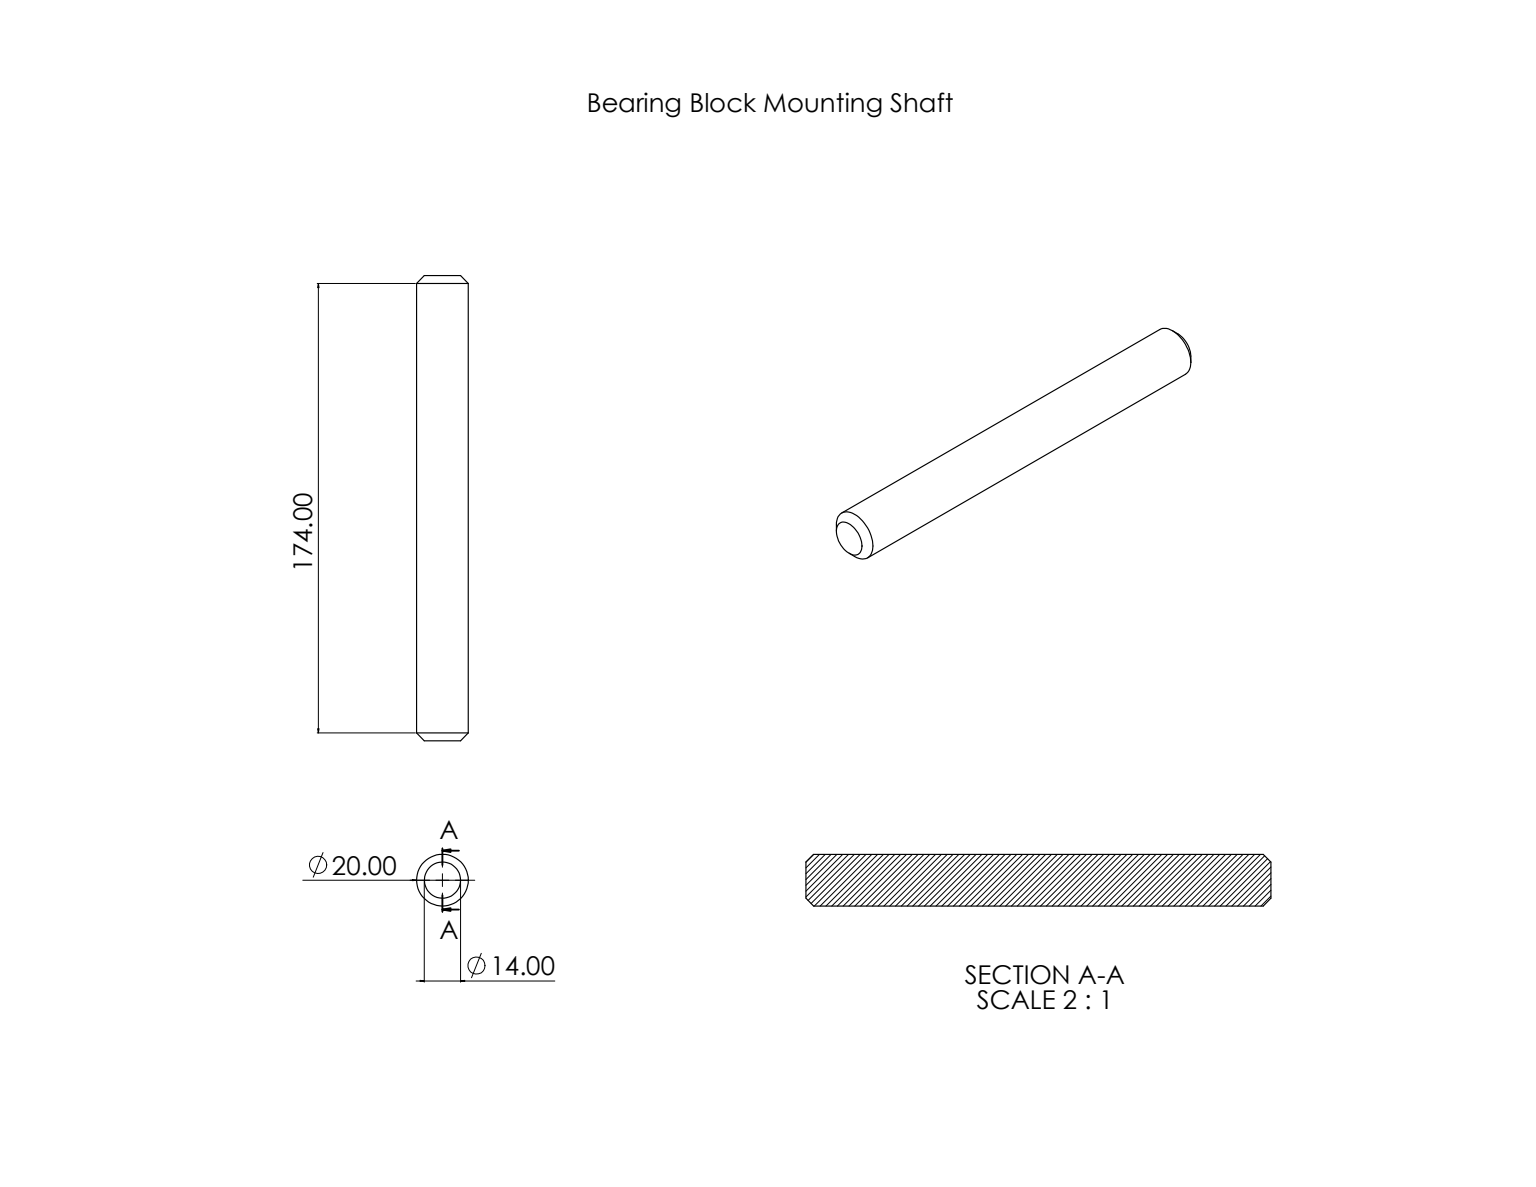
ISO-10303-21;
HEADER;
FILE_DESCRIPTION (('STEP AP214'),
    '1' );
FILE_NAME ('Bearing Block Mounting Shaft.step',
    '2026-10-19T17:36:30',
    ( '' ),
    ( '' ),
    'SwSTEP 2.0',
    'SolidWorks 2025',
    '' );
FILE_SCHEMA (( 'AUTOMOTIVE_DESIGN' ));
ENDSEC;

DATA;
#28=EDGE_CURVE ( 'NONE', #7100, #9959, #2772, .T. ) ;
#57=FACE_OUTER_BOUND ( 'NONE', #633, .T. ) ;
#142=AXIS2_PLACEMENT_3D ( 'NONE', #1198, #5064, #7978 ) ;
#156=DIRECTION ( 'NONE',  ( 1.000000000000000000, 0.000000000000000000, 0.000000000000000000 ) ) ;
#168=DIRECTION ( 'NONE',  ( 0.000000000000000000, -0.000000000000000000, -1.000000000000000000 ) ) ;
#207=DIRECTION ( 'NONE',  ( 1.000000000000000000, 0.000000000000000000, 0.000000000000000000 ) ) ;
#243=EDGE_CURVE ( 'NONE', #9959, #918, #9739, .T. ) ;
#295=DIRECTION ( 'NONE',  ( 1.000000000000000000, 0.000000000000000000, 0.000000000000000000 ) ) ;
#366=ORIENTED_EDGE ( 'NONE', *, *, #12537, .F. ) ;
#595=CIRCLE ( 'NONE', #1008, 10.00000000000000355 ) ;
#633=EDGE_LOOP ( 'NONE', ( #366, #4722, #9019, #2561 ) ) ;
#785=AXIS2_PLACEMENT_3D ( 'NONE', #3854, #7731, #7665 ) ;
#812=PLANE ( 'NONE',  #785 ) ;
#909=( LENGTH_UNIT ( ) NAMED_UNIT ( * ) SI_UNIT ( .MILLI., .METRE. ) );
#918=VERTEX_POINT ( 'NONE', #1888 ) ;
#923=STYLED_ITEM('',(#12584),#10571);
#1001=UNCERTAINTY_MEASURE_WITH_UNIT (LENGTH_MEASURE( 1.000000000000000082E-05 ), #909, 'distance_accuracy_value', 'NONE');
#1008=AXIS2_PLACEMENT_3D ( 'NONE', #4470, #7262, #4286 ) ;
#1021=SHAPE_DEFINITION_REPRESENTATION ( #9949, #1739 ) ;
#1198=CARTESIAN_POINT ( 'NONE',  ( 0.000000000000000000, 20.00000000000000355, 109.9999999999999858 ) ) ;
#1226=DIRECTION ( 'NONE',  ( -0.7071067811865469066, 0.000000000000000000, -0.7071067811865482389 ) ) ;
#1295=DIRECTION ( 'NONE',  ( -0.7071067811865502373, 8.659560562354966138E-17, 0.7071067811865449082 ) ) ;
#1363=ORIENTED_EDGE ( 'NONE', *, *, #3044, .T. ) ;
#1376=ORIENTED_EDGE ( 'NONE', *, *, #2334, .F. ) ;
#1391=ORIENTED_EDGE ( 'NONE', *, *, #2650, .F. ) ;
#1488=AXIS2_PLACEMENT_3D ( 'NONE', #10254, #5256, #5445 ) ;
#1523=EDGE_LOOP ( 'NONE', ( #7715, #1363 ) ) ;
#1633=EDGE_LOOP ( 'NONE', ( #1376, #9658, #7352, #7644 ) ) ;
#1682=DIRECTION ( 'NONE',  ( 1.000000000000000000, 0.000000000000000000, 0.000000000000000000 ) ) ;
#1688=CIRCLE ( 'NONE', #1488, 10.00000000000000355 ) ;
#1693=EDGE_CURVE ( 'NONE', #9959, #2943, #595, .T. ) ;
#1721=APPLICATION_CONTEXT ( 'automotive_design' ) ;
#1739=SHAPE_REPRESENTATION ( 'Bearing Block Mounting Shaft', ( #9021 ), #11237 ) ;
#1777=ORIENTED_EDGE ( 'NONE', *, *, #28, .F. ) ;
#1780=ORIENTED_EDGE ( 'NONE', *, *, #11066, .F. ) ;
#1782=AXIS2_PLACEMENT_3D ( 'NONE', #11582, #168, #295 ) ;
#1878=VERTEX_POINT ( 'NONE', #7643 ) ;
#1888=CARTESIAN_POINT ( 'NONE',  ( 10.00000000000000355, 20.00000000000000355, 106.9999999999999574 ) ) ;
#1955=DIRECTION ( 'NONE',  ( 1.000000000000000000, 0.000000000000000000, 0.000000000000000000 ) ) ;
#2154=CONICAL_SURFACE ( 'NONE', #142, 6.999999999999978684, 0.7853981633974473908 ) ;
#2218=ORIENTED_EDGE ( 'NONE', *, *, #4435, .F. ) ;
#2219=DIRECTION ( 'NONE',  ( 0.7071067811865469066, 8.659560562354926695E-17, -0.7071067811865482389 ) ) ;
#2235=EDGE_CURVE ( 'NONE', #7100, #3380, #7707, .T. ) ;
#2328=CARTESIAN_POINT ( 'NONE',  ( 10.00000000000000355, 20.00000000000000355, -66.99999999999998579 ) ) ;
#2334=EDGE_CURVE ( 'NONE', #3380, #2943, #7056, .T. ) ;
#2472=EDGE_LOOP ( 'NONE', ( #3080, #8282, #4849, #12524 ) ) ;
#2561=ORIENTED_EDGE ( 'NONE', *, *, #2650, .T. ) ;
#2616=VECTOR ( 'NONE', #8531, 1000.000000000000000 ) ;
#2650=EDGE_CURVE ( 'NONE', #918, #9719, #3640, .T. ) ;
#2700=FACE_OUTER_BOUND ( 'NONE', #8576, .T. ) ;
#2727=VECTOR ( 'NONE', #6543, 1000.000000000000000 ) ;
#2744=DIRECTION ( 'NONE',  ( 0.000000000000000000, 0.000000000000000000, 1.000000000000000000 ) ) ;
#2772=LINE ( 'NONE', #2328, #9517 ) ;
#2910=CARTESIAN_POINT ( 'NONE',  ( 0.000000000000000000, 20.00000000000000355, -70.00000000000000000 ) ) ;
#2943=VERTEX_POINT ( 'NONE', #4688 ) ;
#3044=EDGE_CURVE ( 'NONE', #8530, #1878, #4880, .T. ) ;
#3080=ORIENTED_EDGE ( 'NONE', *, *, #1693, .T. ) ;
#3085=DIRECTION ( 'NONE',  ( 0.7071067811865502373, 0.000000000000000000, 0.7071067811865449082 ) ) ;
#3105=ADVANCED_FACE ( 'NONE', ( #57 ), #4878, .T. ) ;
#3203=PRODUCT_DEFINITION_CONTEXT ( 'detailed design', #9995, 'design' ) ;
#3380=VERTEX_POINT ( 'NONE', #8422 ) ;
#3429=ORIENTED_EDGE ( 'NONE', *, *, #2334, .T. ) ;
#3453=FACE_OUTER_BOUND ( 'NONE', #2472, .T. ) ;
#3481=CARTESIAN_POINT ( 'NONE',  ( 6.999999999999978684, 20.00000000000000355, 109.9999999999999858 ) ) ;
#3486=CARTESIAN_POINT ( 'NONE',  ( 0.000000000000000000, 20.00000000000000355, 109.9999999999999858 ) ) ;
#3549=AXIS2_PLACEMENT_3D ( 'NONE', #6623, #4604, #1682 ) ;
#3564=ORIENTED_EDGE ( 'NONE', *, *, #10628, .F. ) ;
#3565=LINE ( 'NONE', #6666, #2727 ) ;
#3640=CIRCLE ( 'NONE', #10729, 10.00000000000000355 ) ;
#3657=ORIENTED_EDGE ( 'NONE', *, *, #4358, .T. ) ;
#3680=EDGE_LOOP ( 'NONE', ( #12031, #12477 ) ) ;
#3741=( GEOMETRIC_REPRESENTATION_CONTEXT ( 3 ) GLOBAL_UNCERTAINTY_ASSIGNED_CONTEXT ( ( #1001 ) ) GLOBAL_UNIT_ASSIGNED_CONTEXT ( ( #909, #4778, #8708 ) ) REPRESENTATION_CONTEXT ( 'NONE', 'WORKASPACE' ) );
#3783=ADVANCED_FACE ( 'NONE', ( #10854 ), #4479, .T. ) ;
#3801=AXIS2_PLACEMENT_3D ( 'NONE', #3486, #12431, #11475 ) ;
#3854=CARTESIAN_POINT ( 'NONE',  ( 0.000000000000000000, 0.000000000000000000, -70.00000000000000000 ) ) ;
#3872=DIRECTION ( 'NONE',  ( 0.000000000000000000, 0.000000000000000000, -1.000000000000000000 ) ) ;
#3876=SHAPE_REPRESENTATION_RELATIONSHIP ( 'NONE' , 'NONE' ,  #1739, #11260 ) ;
#4060=CARTESIAN_POINT ( 'NONE',  ( 0.000000000000000000, 20.00000000000000355, 106.9999999999999574 ) ) ;
#4063=CARTESIAN_POINT ( 'NONE',  ( 0.000000000000000000, 20.00000000000000355, -66.99999999999998579 ) ) ;
#4130=( LENGTH_UNIT ( ) NAMED_UNIT ( * ) SI_UNIT ( .MILLI., .METRE. ) );
#4202=ADVANCED_FACE ( 'NONE', ( #5586 ), #10493, .T. ) ;
#4286=DIRECTION ( 'NONE',  ( 1.000000000000000000, 0.000000000000000000, 0.000000000000000000 ) ) ;
#4357=CARTESIAN_POINT ( 'NONE',  ( 6.999999999999964473, 20.00000000000000355, -70.00000000000000000 ) ) ;
#4358=EDGE_CURVE ( 'NONE', #8530, #918, #11030, .T. ) ;
#4361=CONICAL_SURFACE ( 'NONE', #8417, 10.00000000000000355, 0.7853981633974520538 ) ;
#4397=DIRECTION ( 'NONE',  ( 0.000000000000000000, 0.000000000000000000, 1.000000000000000000 ) ) ;
#4415=FACE_OUTER_BOUND ( 'NONE', #1523, .T. ) ;
#4435=EDGE_CURVE ( 'NONE', #3380, #7100, #5240, .T. ) ;
#4470=CARTESIAN_POINT ( 'NONE',  ( 0.000000000000000000, 20.00000000000000355, -66.99999999999998579 ) ) ;
#4479=CONICAL_SURFACE ( 'NONE', #6106, 10.00000000000000355, 0.7853981633974520538 ) ;
#4601=CIRCLE ( 'NONE', #12299, 6.999999999999978684 ) ;
#4604=DIRECTION ( 'NONE',  ( 0.000000000000000000, 0.000000000000000000, -1.000000000000000000 ) ) ;
#4662=CARTESIAN_POINT ( 'NONE',  ( 10.00000000000000355, 20.00000000000000355, -70.00000000000000000 ) ) ;
#4688=CARTESIAN_POINT ( 'NONE',  ( -10.00000000000000355, 20.00000000000000355, -66.99999999999998579 ) ) ;
#4722=ORIENTED_EDGE ( 'NONE', *, *, #6731, .T. ) ;
#4740=PRODUCT_DEFINITION_FORMATION_WITH_SPECIFIED_SOURCE ( 'ANY', '', #5086, .NOT_KNOWN. ) ;
#4778=( NAMED_UNIT ( * ) PLANE_ANGLE_UNIT ( ) SI_UNIT ( $, .RADIAN. ) );
#4849=ORIENTED_EDGE ( 'NONE', *, *, #11066, .T. ) ;
#4878=CYLINDRICAL_SURFACE ( 'NONE', #5286, 10.00000000000000355 ) ;
#4880=CIRCLE ( 'NONE', #10737, 6.999999999999978684 ) ;
#5026=( NAMED_UNIT ( * ) SI_UNIT ( $, .STERADIAN. ) SOLID_ANGLE_UNIT ( ) );
#5064=DIRECTION ( 'NONE',  ( 0.000000000000000000, 0.000000000000000000, -1.000000000000000000 ) ) ;
#5086=PRODUCT ( 'Bearing Block Mounting Shaft', 'Bearing Block Mounting Shaft', '', ( #9769 ) ) ;
#5216=AXIS2_PLACEMENT_3D ( 'NONE', #8293, #7331, #8044 ) ;
#5240=CIRCLE ( 'NONE', #1782, 6.999999999999964473 ) ;
#5256=DIRECTION ( 'NONE',  ( -0.000000000000000000, -0.000000000000000000, 1.000000000000000000 ) ) ;
#5286=AXIS2_PLACEMENT_3D ( 'NONE', #2910, #8871, #1955 ) ;
#5361=ADVANCED_FACE ( 'NONE', ( #8614 ), #812, .F. ) ;
#5438=PRODUCT_DEFINITION ( 'UNKNOWN', '', #4740, #3203 ) ;
#5445=DIRECTION ( 'NONE',  ( 1.000000000000000000, 0.000000000000000000, 0.000000000000000000 ) ) ;
#5488=VECTOR ( 'NONE', #1295, 1000.000000000000114 ) ;
#5515=CARTESIAN_POINT ( 'NONE',  ( 0.000000000000000000, 20.00000000000000355, 109.9999999999999858 ) ) ;
#5586=FACE_OUTER_BOUND ( 'NONE', #8684, .T. ) ;
#5661=ORIENTED_EDGE ( 'NONE', *, *, #3044, .F. ) ;
#6036=DIRECTION ( 'NONE',  ( -0.000000000000000000, -0.000000000000000000, 1.000000000000000000 ) ) ;
#6063=CLOSED_SHELL ( 'NONE', ( #11041, #9772, #7585, #3105, #5361, #10436, #4202, #3783 ) ) ;
#6106=AXIS2_PLACEMENT_3D ( 'NONE', #4063, #6036, #9910 ) ;
#6169=CARTESIAN_POINT ( 'NONE',  ( -6.999999999999978684, 20.00000000000000355, 109.9999999999999858 ) ) ;
#6543=DIRECTION ( 'NONE',  ( 0.000000000000000000, 0.000000000000000000, 1.000000000000000000 ) ) ;
#6578=DIRECTION ( 'NONE',  ( -0.000000000000000000, 0.000000000000000000, 1.000000000000000000 ) ) ;
#6623=CARTESIAN_POINT ( 'NONE',  ( 0.000000000000000000, 20.00000000000000355, 106.9999999999999574 ) ) ;
#6666=CARTESIAN_POINT ( 'NONE',  ( -10.00000000000000355, 20.00000000000000355, -70.00000000000000000 ) ) ;
#6689=DIRECTION ( 'NONE',  ( 1.000000000000000000, 0.000000000000000000, 0.000000000000000000 ) ) ;
#6731=EDGE_CURVE ( 'NONE', #2943, #9959, #1688, .T. ) ;
#6742=DIRECTION ( 'NONE',  ( 0.000000000000000000, -0.000000000000000000, -1.000000000000000000 ) ) ;
#6922=LINE ( 'NONE', #6169, #10632 ) ;
#7056=LINE ( 'NONE', #9985, #5488 ) ;
#7100=VERTEX_POINT ( 'NONE', #4357 ) ;
#7169=ORIENTED_EDGE ( 'NONE', *, *, #10215, .F. ) ;
#7262=DIRECTION ( 'NONE',  ( -0.000000000000000000, -0.000000000000000000, 1.000000000000000000 ) ) ;
#7331=DIRECTION ( 'NONE',  ( -0.000000000000000000, 0.000000000000000000, 1.000000000000000000 ) ) ;
#7352=ORIENTED_EDGE ( 'NONE', *, *, #28, .T. ) ;
#7482=ORIENTED_EDGE ( 'NONE', *, *, #4358, .F. ) ;
#7585=ADVANCED_FACE ( 'NONE', ( #3453 ), #10120, .T. ) ;
#7643=CARTESIAN_POINT ( 'NONE',  ( -6.999999999999978684, 20.00000000000000355, 109.9999999999999858 ) ) ;
#7644=ORIENTED_EDGE ( 'NONE', *, *, #6731, .F. ) ;
#7665=DIRECTION ( 'NONE',  ( 1.000000000000000000, 0.000000000000000000, 0.000000000000000000 ) ) ;
#7707=CIRCLE ( 'NONE', #8317, 6.999999999999964473 ) ;
#7715=ORIENTED_EDGE ( 'NONE', *, *, #10215, .T. ) ;
#7731=DIRECTION ( 'NONE',  ( -0.000000000000000000, 0.000000000000000000, 1.000000000000000000 ) ) ;
#7800=MECHANICAL_DESIGN_GEOMETRIC_PRESENTATION_REPRESENTATION('',(#923),#3741);
#7938=DIRECTION ( 'NONE',  ( 1.000000000000000000, 0.000000000000000000, 0.000000000000000000 ) ) ;
#7978=DIRECTION ( 'NONE',  ( -1.000000000000000000, 0.000000000000000000, 0.000000000000000000 ) ) ;
#8036=ORIENTED_EDGE ( 'NONE', *, *, #10628, .T. ) ;
#8042=CARTESIAN_POINT ( 'NONE',  ( -10.00000000000000355, 20.00000000000000355, 106.9999999999999574 ) ) ;
#8044=DIRECTION ( 'NONE',  ( 1.000000000000000000, 0.000000000000000000, 0.000000000000000000 ) ) ;
#8116=CARTESIAN_POINT ( 'NONE',  ( 6.999999999999978684, 20.00000000000000355, 109.9999999999999858 ) ) ;
#8195=AXIS2_PLACEMENT_3D ( 'NONE', #12083, #4397, #12144 ) ;
#8282=ORIENTED_EDGE ( 'NONE', *, *, #12537, .T. ) ;
#8293=CARTESIAN_POINT ( 'NONE',  ( 0.000000000000000000, 0.000000000000000000, 109.9999999999999858 ) ) ;
#8317=AXIS2_PLACEMENT_3D ( 'NONE', #9862, #6742, #156 ) ;
#8374=DIRECTION ( 'NONE',  ( 1.000000000000000000, 0.000000000000000000, 0.000000000000000000 ) ) ;
#8417=AXIS2_PLACEMENT_3D ( 'NONE', #9434, #10494, #6689 ) ;
#8422=CARTESIAN_POINT ( 'NONE',  ( -6.999999999999964473, 20.00000000000000355, -70.00000000000000000 ) ) ;
#8497=DIRECTION ( 'NONE',  ( -0.000000000000000000, 0.000000000000000000, 1.000000000000000000 ) ) ;
#8530=VERTEX_POINT ( 'NONE', #3481 ) ;
#8531=DIRECTION ( 'NONE',  ( 0.000000000000000000, 0.000000000000000000, 1.000000000000000000 ) ) ;
#8576=EDGE_LOOP ( 'NONE', ( #2218, #3429, #10393, #1777 ) ) ;
#8614=FACE_OUTER_BOUND ( 'NONE', #3680, .T. ) ;
#8684=EDGE_LOOP ( 'NONE', ( #7482, #7169, #8036, #1391 ) ) ;
#8686=UNCERTAINTY_MEASURE_WITH_UNIT (LENGTH_MEASURE( 1.000000000000000082E-05 ), #4130, 'distance_accuracy_value', 'NONE');
#8708=( NAMED_UNIT ( * ) SI_UNIT ( $, .STERADIAN. ) SOLID_ANGLE_UNIT ( ) );
#8871=DIRECTION ( 'NONE',  ( 0.000000000000000000, 0.000000000000000000, 1.000000000000000000 ) ) ;
#9019=ORIENTED_EDGE ( 'NONE', *, *, #243, .T. ) ;
#9021=AXIS2_PLACEMENT_3D ( 'NONE', #11433, #2744, #207 ) ;
#9031=CIRCLE ( 'NONE', #3549, 10.00000000000000355 ) ;
#9049=EDGE_LOOP ( 'NONE', ( #5661, #3657, #1780, #3564 ) ) ;
#9434=CARTESIAN_POINT ( 'NONE',  ( 0.000000000000000000, 20.00000000000000355, -66.99999999999998579 ) ) ;
#9517=VECTOR ( 'NONE', #3085, 1000.000000000000114 ) ;
#9658=ORIENTED_EDGE ( 'NONE', *, *, #2235, .F. ) ;
#9719=VERTEX_POINT ( 'NONE', #8042 ) ;
#9739=LINE ( 'NONE', #4662, #2616 ) ;
#9769=PRODUCT_CONTEXT ( 'NONE', #1721, 'mechanical' ) ;
#9772=ADVANCED_FACE ( 'NONE', ( #9885 ), #2154, .T. ) ;
#9862=CARTESIAN_POINT ( 'NONE',  ( 0.000000000000000000, 20.00000000000000355, -70.00000000000000000 ) ) ;
#9885=FACE_OUTER_BOUND ( 'NONE', #9049, .T. ) ;
#9910=DIRECTION ( 'NONE',  ( 1.000000000000000000, 0.000000000000000000, 0.000000000000000000 ) ) ;
#9949=PRODUCT_DEFINITION_SHAPE ( 'NONE', 'NONE',  #5438 ) ;
#9959=VERTEX_POINT ( 'NONE', #11093 ) ;
#9985=CARTESIAN_POINT ( 'NONE',  ( -10.00000000000000355, 20.00000000000000355, -66.99999999999998579 ) ) ;
#9995=APPLICATION_CONTEXT ( 'automotive_design' ) ;
#10120=CYLINDRICAL_SURFACE ( 'NONE', #8195, 10.00000000000000355 ) ;
#10215=EDGE_CURVE ( 'NONE', #1878, #8530, #4601, .T. ) ;
#10254=CARTESIAN_POINT ( 'NONE',  ( 0.000000000000000000, 20.00000000000000355, -66.99999999999998579 ) ) ;
#10269=CARTESIAN_POINT ( 'NONE',  ( 0.000000000000000000, 20.00000000000000355, 109.9999999999999858 ) ) ;
#10393=ORIENTED_EDGE ( 'NONE', *, *, #1693, .F. ) ;
#10436=ADVANCED_FACE ( 'NONE', ( #4415 ), #11141, .T. ) ;
#10442=DIRECTION ( 'NONE',  ( 1.000000000000000000, 0.000000000000000000, 0.000000000000000000 ) ) ;
#10493=CONICAL_SURFACE ( 'NONE', #3801, 6.999999999999978684, 0.7853981633974473908 ) ;
#10494=DIRECTION ( 'NONE',  ( -0.000000000000000000, -0.000000000000000000, 1.000000000000000000 ) ) ;
#10571=MANIFOLD_SOLID_BREP ( 'Chamfer3', #6063 ) ;
#10628=EDGE_CURVE ( 'NONE', #1878, #9719, #6922, .T. ) ;
#10632=VECTOR ( 'NONE', #1226, 999.9999999999998863 ) ;
#10729=AXIS2_PLACEMENT_3D ( 'NONE', #4060, #3872, #7938 ) ;
#10737=AXIS2_PLACEMENT_3D ( 'NONE', #10269, #8497, #8374 ) ;
#10854=FACE_OUTER_BOUND ( 'NONE', #1633, .T. ) ;
#11030=LINE ( 'NONE', #8116, #11310 ) ;
#11041=ADVANCED_FACE ( 'NONE', ( #2700 ), #4361, .T. ) ;
#11066=EDGE_CURVE ( 'NONE', #9719, #918, #9031, .T. ) ;
#11093=CARTESIAN_POINT ( 'NONE',  ( 10.00000000000000355, 20.00000000000000355, -66.99999999999998579 ) ) ;
#11141=PLANE ( 'NONE',  #5216 ) ;
#11237=( GEOMETRIC_REPRESENTATION_CONTEXT ( 3 ) GLOBAL_UNCERTAINTY_ASSIGNED_CONTEXT ( ( #8686 ) ) GLOBAL_UNIT_ASSIGNED_CONTEXT ( ( #4130, #11620, #5026 ) ) REPRESENTATION_CONTEXT ( 'NONE', 'WORKASPACE' ) );
#11260=ADVANCED_BREP_SHAPE_REPRESENTATION ( '', ( #10571, #9021 ), #11237 ) ;
#11310=VECTOR ( 'NONE', #2219, 999.9999999999998863 ) ;
#11433=CARTESIAN_POINT ( 'NONE',  ( 0.000000000000000000, 0.000000000000000000, 0.000000000000000000 ) ) ;
#11475=DIRECTION ( 'NONE',  ( -1.000000000000000000, 0.000000000000000000, 0.000000000000000000 ) ) ;
#11582=CARTESIAN_POINT ( 'NONE',  ( 0.000000000000000000, 20.00000000000000355, -70.00000000000000000 ) ) ;
#11620=( NAMED_UNIT ( * ) PLANE_ANGLE_UNIT ( ) SI_UNIT ( $, .RADIAN. ) );
#12031=ORIENTED_EDGE ( 'NONE', *, *, #2235, .T. ) ;
#12083=CARTESIAN_POINT ( 'NONE',  ( 0.000000000000000000, 20.00000000000000355, -70.00000000000000000 ) ) ;
#12144=DIRECTION ( 'NONE',  ( 1.000000000000000000, 0.000000000000000000, 0.000000000000000000 ) ) ;
#12299=AXIS2_PLACEMENT_3D ( 'NONE', #5515, #6578, #10442 ) ;
#12431=DIRECTION ( 'NONE',  ( 0.000000000000000000, 0.000000000000000000, -1.000000000000000000 ) ) ;
#12477=ORIENTED_EDGE ( 'NONE', *, *, #4435, .T. ) ;
#12524=ORIENTED_EDGE ( 'NONE', *, *, #243, .F. ) ;
#12537=EDGE_CURVE ( 'NONE', #2943, #9719, #3565, .T. ) ;
#12578=COLOUR_RGB('Grey',0.48,0.52,0.57);
#12579=FILL_AREA_STYLE_COLOUR('',#12578);
#12580=FILL_AREA_STYLE('',(#12579));
#12581=SURFACE_STYLE_FILL_AREA(#12580);
#12582=SURFACE_SIDE_STYLE('',(#12581));
#12583=SURFACE_STYLE_USAGE(.BOTH.,#12582);
#12584=PRESENTATION_STYLE_ASSIGNMENT((#12583));
ENDSEC;
END-ISO-10303-21;
